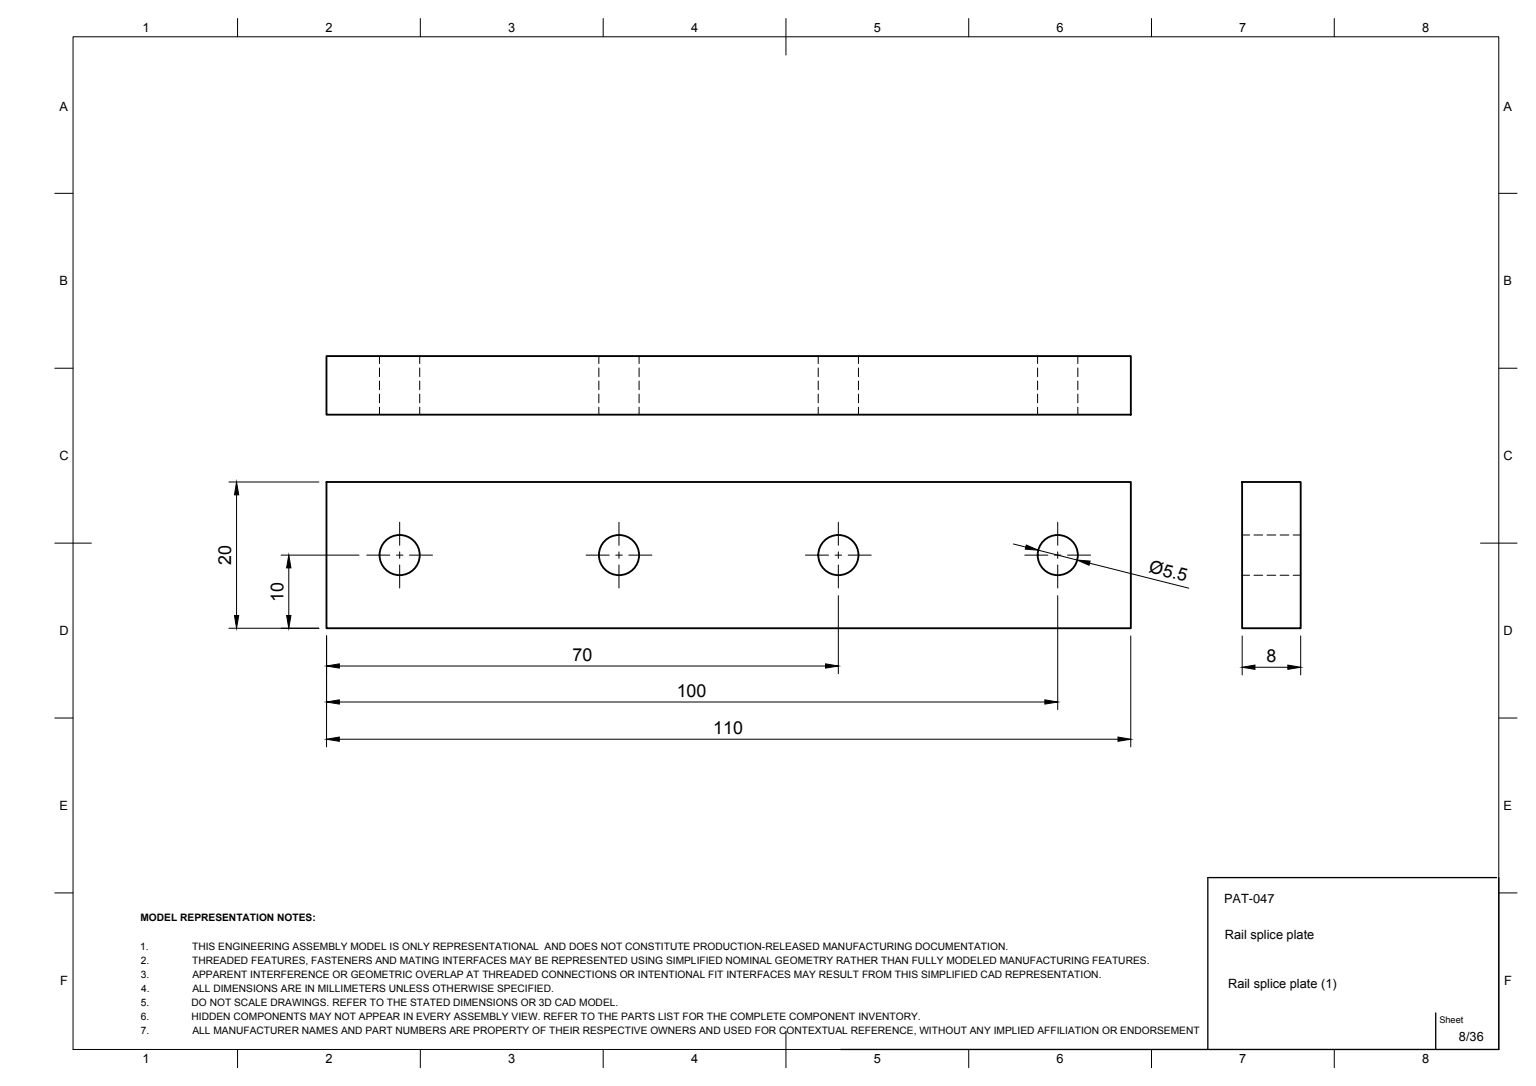
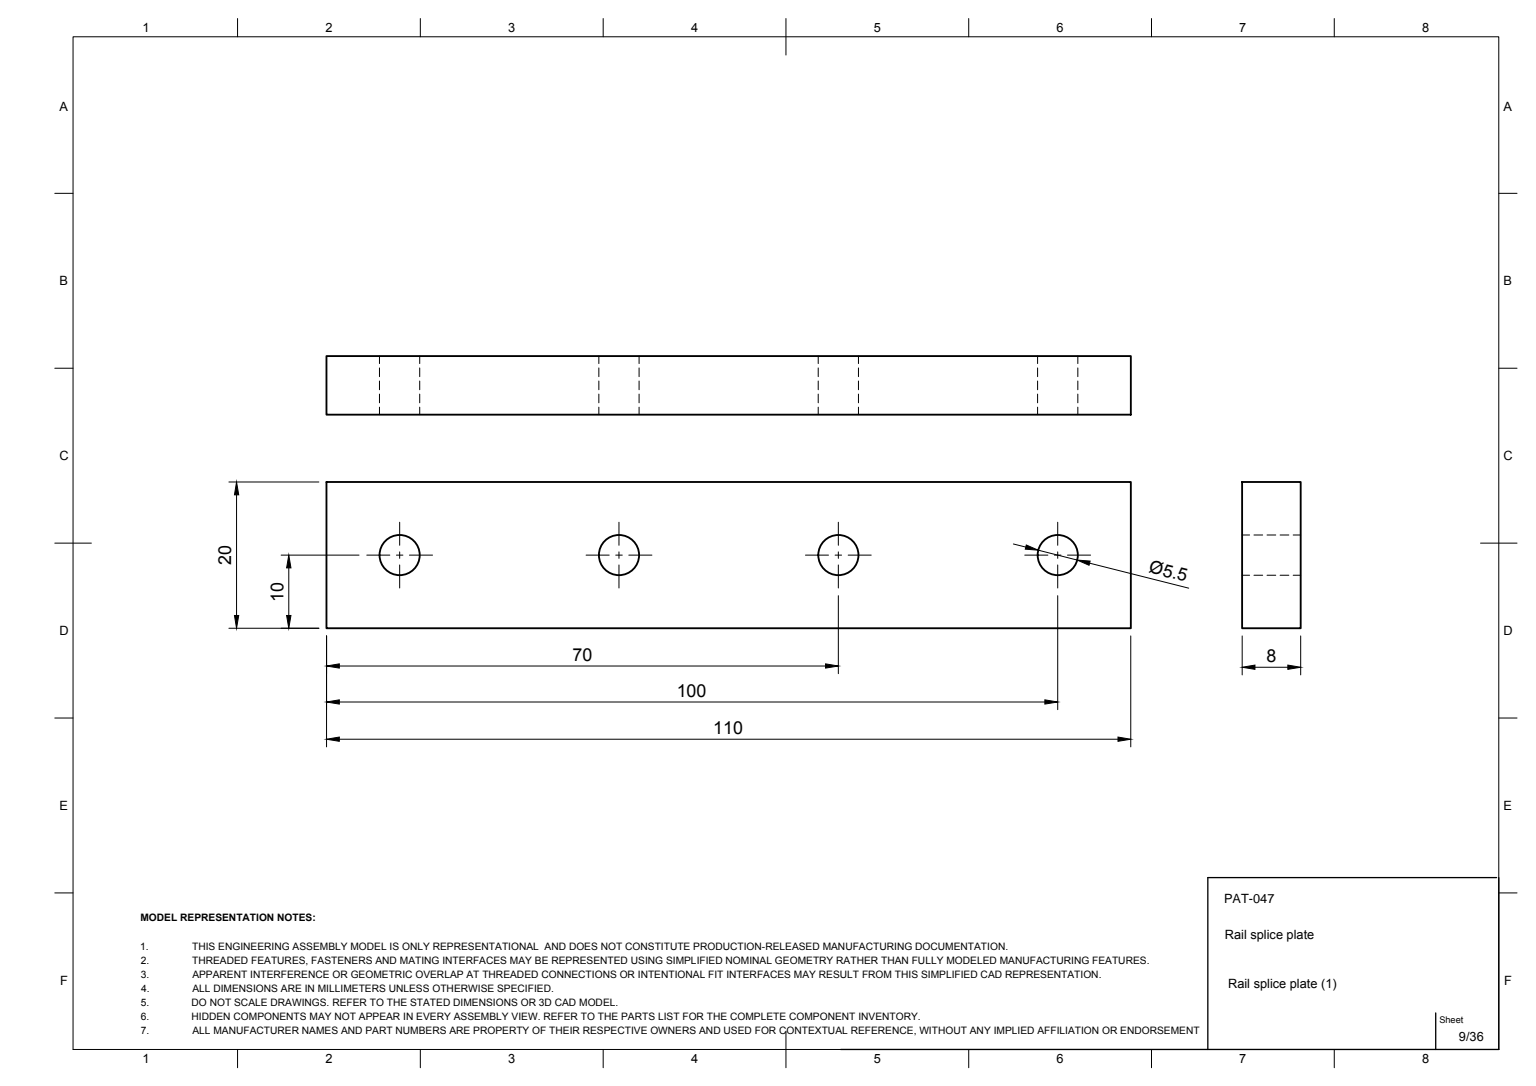
ISO-10303-21;
HEADER;
/* Generated by software containing ST-Developer
 * from STEP Tools, Inc. (www.steptools.com) 
 */

FILE_DESCRIPTION(
/* description */ ('Gravity roller conveyor section'),
/* implementation_level */ '2;1');

FILE_NAME(
/* name */ 'Rail splice plate.step',
/* time_stamp */ '2026-11-02T07:43:02-08:00',
/* author */ (''),
/* organization */ (''),
/* preprocessor_version */ 'ST-DEVELOPER v20.2',
/* originating_system */ 'Autodesk Translation Framework v15.17.0.0',
/* authorisation */ '');

FILE_SCHEMA (('AUTOMOTIVE_DESIGN { 1 0 10303 214 3 1 1 }'));
ENDSEC;

DATA;
#10=MECHANICAL_DESIGN_GEOMETRIC_PRESENTATION_REPRESENTATION('',(#529),#13821);
#461=SHAPE_REPRESENTATION_RELATIONSHIP('SRR','None',#13998,#495);
#495=ADVANCED_BREP_SHAPE_REPRESENTATION('',(#571),#13785);
#529=STYLED_ITEM('',(#14191),#571);
#571=MANIFOLD_SOLID_BREP('Body1',#7627);
#609=FACE_BOUND('',#1431,.T.);
#610=FACE_BOUND('',#1432,.T.);
#611=FACE_BOUND('',#1433,.T.);
#612=FACE_BOUND('',#1434,.T.);
#613=FACE_BOUND('',#1437,.T.);
#614=FACE_BOUND('',#1438,.T.);
#615=FACE_BOUND('',#1439,.T.);
#616=FACE_BOUND('',#1440,.T.);
#702=PLANE('',#8063);
#703=PLANE('',#8064);
#704=PLANE('',#8065);
#705=PLANE('',#8066);
#706=PLANE('',#8067);
#707=PLANE('',#8068);
#1007=FACE_OUTER_BOUND('',#1426,.T.);
#1008=FACE_OUTER_BOUND('',#1427,.T.);
#1009=FACE_OUTER_BOUND('',#1428,.T.);
#1010=FACE_OUTER_BOUND('',#1429,.T.);
#1011=FACE_OUTER_BOUND('',#1430,.T.);
#1012=FACE_OUTER_BOUND('',#1435,.T.);
#1013=FACE_OUTER_BOUND('',#1436,.T.);
#1014=FACE_OUTER_BOUND('',#1441,.T.);
#1015=FACE_OUTER_BOUND('',#1442,.T.);
#1016=FACE_OUTER_BOUND('',#1443,.T.);
#1426=EDGE_LOOP('',(#5202,#5203,#5204,#5205));
#1427=EDGE_LOOP('',(#5206,#5207,#5208,#5209));
#1428=EDGE_LOOP('',(#5210,#5211,#5212,#5213));
#1429=EDGE_LOOP('',(#5214,#5215,#5216,#5217));
#1430=EDGE_LOOP('',(#5218,#5219,#5220,#5221));
#1431=EDGE_LOOP('',(#5222));
#1432=EDGE_LOOP('',(#5223));
#1433=EDGE_LOOP('',(#5224));
#1434=EDGE_LOOP('',(#5225));
#1435=EDGE_LOOP('',(#5226,#5227,#5228,#5229));
#1436=EDGE_LOOP('',(#5230,#5231,#5232,#5233));
#1437=EDGE_LOOP('',(#5234));
#1438=EDGE_LOOP('',(#5235));
#1439=EDGE_LOOP('',(#5236));
#1440=EDGE_LOOP('',(#5237));
#1441=EDGE_LOOP('',(#5238,#5239,#5240,#5241));
#1442=EDGE_LOOP('',(#5242,#5243,#5244,#5245));
#1443=EDGE_LOOP('',(#5246,#5247,#5248,#5249));
#1938=LINE('',#11080,#2656);
#1939=LINE('',#11086,#2657);
#1940=LINE('',#11092,#2658);
#1941=LINE('',#11098,#2659);
#1942=LINE('',#11103,#2660);
#1943=LINE('',#11105,#2661);
#1944=LINE('',#11107,#2662);
#1945=LINE('',#11108,#2663);
#1946=LINE('',#11111,#2664);
#1947=LINE('',#11113,#2665);
#1948=LINE('',#11114,#2666);
#1949=LINE('',#11117,#2667);
#1950=LINE('',#11119,#2668);
#1951=LINE('',#11120,#2669);
#1952=LINE('',#11122,#2670);
#1953=LINE('',#11123,#2671);
#2656=VECTOR('',#8827,0.274999999999999);
#2657=VECTOR('',#8834,0.274999999999999);
#2658=VECTOR('',#8841,0.274999999999999);
#2659=VECTOR('',#8848,0.274999999999999);
#2660=VECTOR('',#8853,1.);
#2661=VECTOR('',#8854,1.);
#2662=VECTOR('',#8855,1.);
#2663=VECTOR('',#8856,1.);
#2664=VECTOR('',#8859,1.);
#2665=VECTOR('',#8860,1.);
#2666=VECTOR('',#8861,1.);
#2667=VECTOR('',#8864,1.);
#2668=VECTOR('',#8865,1.);
#2669=VECTOR('',#8866,1.);
#2670=VECTOR('',#8869,1.);
#2671=VECTOR('',#8870,1.);
#3374=CIRCLE('',#8052,0.274999999999999);
#3375=CIRCLE('',#8053,0.274999999999999);
#3376=CIRCLE('',#8055,0.274999999999999);
#3377=CIRCLE('',#8056,0.274999999999999);
#3378=CIRCLE('',#8058,0.274999999999999);
#3379=CIRCLE('',#8059,0.274999999999999);
#3380=CIRCLE('',#8061,0.274999999999999);
#3381=CIRCLE('',#8062,0.274999999999999);
#3590=VERTEX_POINT('',#11077);
#3591=VERTEX_POINT('',#11079);
#3592=VERTEX_POINT('',#11083);
#3593=VERTEX_POINT('',#11085);
#3594=VERTEX_POINT('',#11089);
#3595=VERTEX_POINT('',#11091);
#3596=VERTEX_POINT('',#11095);
#3597=VERTEX_POINT('',#11097);
#3598=VERTEX_POINT('',#11101);
#3599=VERTEX_POINT('',#11102);
#3600=VERTEX_POINT('',#11104);
#3601=VERTEX_POINT('',#11106);
#3602=VERTEX_POINT('',#11110);
#3603=VERTEX_POINT('',#11112);
#3604=VERTEX_POINT('',#11116);
#3605=VERTEX_POINT('',#11118);
#4238=EDGE_CURVE('',#3590,#3590,#3374,.T.);
#4239=EDGE_CURVE('',#3590,#3591,#1938,.T.);
#4240=EDGE_CURVE('',#3591,#3591,#3375,.T.);
#4241=EDGE_CURVE('',#3592,#3592,#3376,.T.);
#4242=EDGE_CURVE('',#3592,#3593,#1939,.T.);
#4243=EDGE_CURVE('',#3593,#3593,#3377,.T.);
#4244=EDGE_CURVE('',#3594,#3594,#3378,.T.);
#4245=EDGE_CURVE('',#3594,#3595,#1940,.T.);
#4246=EDGE_CURVE('',#3595,#3595,#3379,.T.);
#4247=EDGE_CURVE('',#3596,#3596,#3380,.T.);
#4248=EDGE_CURVE('',#3596,#3597,#1941,.T.);
#4249=EDGE_CURVE('',#3597,#3597,#3381,.T.);
#4250=EDGE_CURVE('',#3598,#3599,#1942,.T.);
#4251=EDGE_CURVE('',#3599,#3600,#1943,.T.);
#4252=EDGE_CURVE('',#3601,#3600,#1944,.T.);
#4253=EDGE_CURVE('',#3598,#3601,#1945,.T.);
#4254=EDGE_CURVE('',#3602,#3598,#1946,.T.);
#4255=EDGE_CURVE('',#3603,#3601,#1947,.T.);
#4256=EDGE_CURVE('',#3602,#3603,#1948,.T.);
#4257=EDGE_CURVE('',#3604,#3602,#1949,.T.);
#4258=EDGE_CURVE('',#3605,#3603,#1950,.T.);
#4259=EDGE_CURVE('',#3604,#3605,#1951,.T.);
#4260=EDGE_CURVE('',#3599,#3604,#1952,.T.);
#4261=EDGE_CURVE('',#3600,#3605,#1953,.T.);
#5202=ORIENTED_EDGE('',*,*,#4238,.F.);
#5203=ORIENTED_EDGE('',*,*,#4239,.T.);
#5204=ORIENTED_EDGE('',*,*,#4240,.F.);
#5205=ORIENTED_EDGE('',*,*,#4239,.F.);
#5206=ORIENTED_EDGE('',*,*,#4241,.F.);
#5207=ORIENTED_EDGE('',*,*,#4242,.T.);
#5208=ORIENTED_EDGE('',*,*,#4243,.F.);
#5209=ORIENTED_EDGE('',*,*,#4242,.F.);
#5210=ORIENTED_EDGE('',*,*,#4244,.F.);
#5211=ORIENTED_EDGE('',*,*,#4245,.T.);
#5212=ORIENTED_EDGE('',*,*,#4246,.F.);
#5213=ORIENTED_EDGE('',*,*,#4245,.F.);
#5214=ORIENTED_EDGE('',*,*,#4247,.F.);
#5215=ORIENTED_EDGE('',*,*,#4248,.T.);
#5216=ORIENTED_EDGE('',*,*,#4249,.F.);
#5217=ORIENTED_EDGE('',*,*,#4248,.F.);
#5218=ORIENTED_EDGE('',*,*,#4250,.T.);
#5219=ORIENTED_EDGE('',*,*,#4251,.T.);
#5220=ORIENTED_EDGE('',*,*,#4252,.F.);
#5221=ORIENTED_EDGE('',*,*,#4253,.F.);
#5222=ORIENTED_EDGE('',*,*,#4240,.T.);
#5223=ORIENTED_EDGE('',*,*,#4243,.T.);
#5224=ORIENTED_EDGE('',*,*,#4246,.T.);
#5225=ORIENTED_EDGE('',*,*,#4249,.T.);
#5226=ORIENTED_EDGE('',*,*,#4254,.T.);
#5227=ORIENTED_EDGE('',*,*,#4253,.T.);
#5228=ORIENTED_EDGE('',*,*,#4255,.F.);
#5229=ORIENTED_EDGE('',*,*,#4256,.F.);
#5230=ORIENTED_EDGE('',*,*,#4257,.T.);
#5231=ORIENTED_EDGE('',*,*,#4256,.T.);
#5232=ORIENTED_EDGE('',*,*,#4258,.F.);
#5233=ORIENTED_EDGE('',*,*,#4259,.F.);
#5234=ORIENTED_EDGE('',*,*,#4238,.T.);
#5235=ORIENTED_EDGE('',*,*,#4241,.T.);
#5236=ORIENTED_EDGE('',*,*,#4244,.T.);
#5237=ORIENTED_EDGE('',*,*,#4247,.T.);
#5238=ORIENTED_EDGE('',*,*,#4260,.T.);
#5239=ORIENTED_EDGE('',*,*,#4259,.T.);
#5240=ORIENTED_EDGE('',*,*,#4261,.F.);
#5241=ORIENTED_EDGE('',*,*,#4251,.F.);
#5242=ORIENTED_EDGE('',*,*,#4261,.T.);
#5243=ORIENTED_EDGE('',*,*,#4258,.T.);
#5244=ORIENTED_EDGE('',*,*,#4255,.T.);
#5245=ORIENTED_EDGE('',*,*,#4252,.T.);
#5246=ORIENTED_EDGE('',*,*,#4260,.F.);
#5247=ORIENTED_EDGE('',*,*,#4250,.F.);
#5248=ORIENTED_EDGE('',*,*,#4254,.F.);
#5249=ORIENTED_EDGE('',*,*,#4257,.F.);
#7130=CYLINDRICAL_SURFACE('',#8051,0.274999999999999);
#7131=CYLINDRICAL_SURFACE('',#8054,0.274999999999999);
#7132=CYLINDRICAL_SURFACE('',#8057,0.274999999999999);
#7133=CYLINDRICAL_SURFACE('',#8060,0.274999999999999);
#7208=ADVANCED_FACE('',(#1007),#7130,.F.);
#7209=ADVANCED_FACE('',(#1008),#7131,.F.);
#7210=ADVANCED_FACE('',(#1009),#7132,.F.);
#7211=ADVANCED_FACE('',(#1010),#7133,.F.);
#7212=ADVANCED_FACE('',(#1011,#609,#610,#611,#612),#702,.T.);
#7213=ADVANCED_FACE('',(#1012),#703,.T.);
#7214=ADVANCED_FACE('',(#1013,#613,#614,#615,#616),#704,.T.);
#7215=ADVANCED_FACE('',(#1014),#705,.T.);
#7216=ADVANCED_FACE('',(#1015),#706,.T.);
#7217=ADVANCED_FACE('',(#1016),#707,.F.);
#7627=CLOSED_SHELL('',(#7208,#7209,#7210,#7211,#7212,#7213,#7214,#7215,
#7216,#7217));
#8050=AXIS2_PLACEMENT_3D('',#11075,#8821,#8822);
#8051=AXIS2_PLACEMENT_3D('',#11076,#8823,#8824);
#8052=AXIS2_PLACEMENT_3D('',#11078,#8825,#8826);
#8053=AXIS2_PLACEMENT_3D('',#11081,#8828,#8829);
#8054=AXIS2_PLACEMENT_3D('',#11082,#8830,#8831);
#8055=AXIS2_PLACEMENT_3D('',#11084,#8832,#8833);
#8056=AXIS2_PLACEMENT_3D('',#11087,#8835,#8836);
#8057=AXIS2_PLACEMENT_3D('',#11088,#8837,#8838);
#8058=AXIS2_PLACEMENT_3D('',#11090,#8839,#8840);
#8059=AXIS2_PLACEMENT_3D('',#11093,#8842,#8843);
#8060=AXIS2_PLACEMENT_3D('',#11094,#8844,#8845);
#8061=AXIS2_PLACEMENT_3D('',#11096,#8846,#8847);
#8062=AXIS2_PLACEMENT_3D('',#11099,#8849,#8850);
#8063=AXIS2_PLACEMENT_3D('',#11100,#8851,#8852);
#8064=AXIS2_PLACEMENT_3D('',#11109,#8857,#8858);
#8065=AXIS2_PLACEMENT_3D('',#11115,#8862,#8863);
#8066=AXIS2_PLACEMENT_3D('',#11121,#8867,#8868);
#8067=AXIS2_PLACEMENT_3D('',#11124,#8871,#8872);
#8068=AXIS2_PLACEMENT_3D('',#11125,#8873,#8874);
#8821=DIRECTION('axis',(0.,0.,1.));
#8822=DIRECTION('refdir',(1.,0.,0.));
#8823=DIRECTION('center_axis',(0.,1.,0.));
#8824=DIRECTION('ref_axis',(1.,0.,0.));
#8825=DIRECTION('center_axis',(0.,1.,0.));
#8826=DIRECTION('ref_axis',(1.,0.,0.));
#8827=DIRECTION('',(0.,1.,0.));
#8828=DIRECTION('center_axis',(0.,-1.,0.));
#8829=DIRECTION('ref_axis',(1.,0.,0.));
#8830=DIRECTION('center_axis',(0.,1.,0.));
#8831=DIRECTION('ref_axis',(1.,0.,0.));
#8832=DIRECTION('center_axis',(0.,1.,0.));
#8833=DIRECTION('ref_axis',(1.,0.,0.));
#8834=DIRECTION('',(0.,1.,0.));
#8835=DIRECTION('center_axis',(0.,-1.,0.));
#8836=DIRECTION('ref_axis',(1.,0.,0.));
#8837=DIRECTION('center_axis',(0.,1.,0.));
#8838=DIRECTION('ref_axis',(1.,0.,0.));
#8839=DIRECTION('center_axis',(0.,1.,0.));
#8840=DIRECTION('ref_axis',(1.,0.,0.));
#8841=DIRECTION('',(0.,1.,0.));
#8842=DIRECTION('center_axis',(0.,-1.,0.));
#8843=DIRECTION('ref_axis',(1.,0.,0.));
#8844=DIRECTION('center_axis',(0.,1.,0.));
#8845=DIRECTION('ref_axis',(1.,0.,0.));
#8846=DIRECTION('center_axis',(0.,1.,0.));
#8847=DIRECTION('ref_axis',(1.,0.,0.));
#8848=DIRECTION('',(0.,1.,0.));
#8849=DIRECTION('center_axis',(0.,-1.,0.));
#8850=DIRECTION('ref_axis',(1.,0.,0.));
#8851=DIRECTION('center_axis',(0.,1.,0.));
#8852=DIRECTION('ref_axis',(-1.,0.,0.));
#8853=DIRECTION('',(-1.,0.,0.));
#8854=DIRECTION('',(0.,0.,1.));
#8855=DIRECTION('',(-1.,0.,0.));
#8856=DIRECTION('',(0.,0.,1.));
#8857=DIRECTION('center_axis',(1.,0.,0.));
#8858=DIRECTION('ref_axis',(0.,1.,0.));
#8859=DIRECTION('',(0.,1.,0.));
#8860=DIRECTION('',(0.,1.,0.));
#8861=DIRECTION('',(0.,0.,1.));
#8862=DIRECTION('center_axis',(0.,-1.,0.));
#8863=DIRECTION('ref_axis',(1.,0.,0.));
#8864=DIRECTION('',(1.,0.,0.));
#8865=DIRECTION('',(1.,0.,0.));
#8866=DIRECTION('',(0.,0.,1.));
#8867=DIRECTION('center_axis',(-1.,0.,0.));
#8868=DIRECTION('ref_axis',(0.,-1.,0.));
#8869=DIRECTION('',(0.,-1.,0.));
#8870=DIRECTION('',(0.,-1.,0.));
#8871=DIRECTION('center_axis',(0.,0.,1.));
#8872=DIRECTION('ref_axis',(1.,0.,0.));
#8873=DIRECTION('center_axis',(0.,0.,1.));
#8874=DIRECTION('ref_axis',(1.,0.,0.));
#11075=CARTESIAN_POINT('',(0.,0.,0.));
#11076=CARTESIAN_POINT('Origin',(42.,-3.9,5.));
#11077=CARTESIAN_POINT('',(41.725,-3.8,5.));
#11078=CARTESIAN_POINT('Origin',(42.,-3.8,5.));
#11079=CARTESIAN_POINT('',(41.725,-3.,5.));
#11080=CARTESIAN_POINT('',(41.725,-3.9,5.));
#11081=CARTESIAN_POINT('Origin',(42.,-3.,5.));
#11082=CARTESIAN_POINT('Origin',(39.,-3.9,5.));
#11083=CARTESIAN_POINT('',(38.725,-3.8,5.));
#11084=CARTESIAN_POINT('Origin',(39.,-3.8,5.));
#11085=CARTESIAN_POINT('',(38.725,-3.,5.));
#11086=CARTESIAN_POINT('',(38.725,-3.9,5.));
#11087=CARTESIAN_POINT('Origin',(39.,-3.,5.));
#11088=CARTESIAN_POINT('Origin',(36.,-3.9,5.));
#11089=CARTESIAN_POINT('',(35.725,-3.8,5.));
#11090=CARTESIAN_POINT('Origin',(36.,-3.8,5.));
#11091=CARTESIAN_POINT('',(35.725,-3.,5.));
#11092=CARTESIAN_POINT('',(35.725,-3.9,5.));
#11093=CARTESIAN_POINT('Origin',(36.,-3.,5.));
#11094=CARTESIAN_POINT('Origin',(45.,-3.9,5.));
#11095=CARTESIAN_POINT('',(44.725,-3.8,5.));
#11096=CARTESIAN_POINT('Origin',(45.,-3.8,5.));
#11097=CARTESIAN_POINT('',(44.725,-3.,5.));
#11098=CARTESIAN_POINT('',(44.725,-3.9,5.));
#11099=CARTESIAN_POINT('Origin',(45.,-3.,5.));
#11100=CARTESIAN_POINT('Origin',(46.,-3.,4.));
#11101=CARTESIAN_POINT('',(46.,-3.,4.));
#11102=CARTESIAN_POINT('',(35.,-3.,4.));
#11103=CARTESIAN_POINT('',(46.,-3.,4.));
#11104=CARTESIAN_POINT('',(35.,-3.,6.));
#11105=CARTESIAN_POINT('',(35.,-3.,4.));
#11106=CARTESIAN_POINT('',(46.,-3.,6.));
#11107=CARTESIAN_POINT('',(46.,-3.,6.));
#11108=CARTESIAN_POINT('',(46.,-3.,4.));
#11109=CARTESIAN_POINT('Origin',(46.,-3.8,4.));
#11110=CARTESIAN_POINT('',(46.,-3.8,4.));
#11111=CARTESIAN_POINT('',(46.,-3.8,4.));
#11112=CARTESIAN_POINT('',(46.,-3.8,6.));
#11113=CARTESIAN_POINT('',(46.,-3.8,6.));
#11114=CARTESIAN_POINT('',(46.,-3.8,4.));
#11115=CARTESIAN_POINT('Origin',(35.,-3.8,4.));
#11116=CARTESIAN_POINT('',(35.,-3.8,4.));
#11117=CARTESIAN_POINT('',(35.,-3.8,4.));
#11118=CARTESIAN_POINT('',(35.,-3.8,6.));
#11119=CARTESIAN_POINT('',(35.,-3.8,6.));
#11120=CARTESIAN_POINT('',(35.,-3.8,4.));
#11121=CARTESIAN_POINT('Origin',(35.,-3.,4.));
#11122=CARTESIAN_POINT('',(35.,-3.,4.));
#11123=CARTESIAN_POINT('',(35.,-3.,6.));
#11124=CARTESIAN_POINT('Origin',(40.5,-3.4,6.));
#11125=CARTESIAN_POINT('Origin',(40.5,-3.4,4.));
#13746=UNCERTAINTY_MEASURE_WITH_UNIT(LENGTH_MEASURE(0.001),#13822,
'DISTANCE_ACCURACY_VALUE',
'Maximum model space distance between geometric entities at asserted c
onnectivities');
#13782=UNCERTAINTY_MEASURE_WITH_UNIT(LENGTH_MEASURE(0.001),#13822,
'DISTANCE_ACCURACY_VALUE',
'Maximum model space distance between geometric entities at asserted c
onnectivities');
#13785=(
GEOMETRIC_REPRESENTATION_CONTEXT(3)
GLOBAL_UNCERTAINTY_ASSIGNED_CONTEXT((#13746))
GLOBAL_UNIT_ASSIGNED_CONTEXT((#13822,#13824,#13825))
REPRESENTATION_CONTEXT('','3D')
);
#13821=(
GEOMETRIC_REPRESENTATION_CONTEXT(3)
GLOBAL_UNCERTAINTY_ASSIGNED_CONTEXT((#13782))
GLOBAL_UNIT_ASSIGNED_CONTEXT((#13822,#13824,#13825))
REPRESENTATION_CONTEXT('','3D')
);
#13822=(
LENGTH_UNIT()
NAMED_UNIT(*)
SI_UNIT(.CENTI.,.METRE.)
);
#13824=(
NAMED_UNIT(*)
PLANE_ANGLE_UNIT()
SI_UNIT($,.RADIAN.)
);
#13825=(
NAMED_UNIT(*)
SI_UNIT($,.STERADIAN.)
SOLID_ANGLE_UNIT()
);
#13828=SHAPE_DEFINITION_REPRESENTATION(#13866,#13998);
#13866=PRODUCT_DEFINITION_SHAPE('',$,#14037);
#13998=SHAPE_REPRESENTATION('',(#8050),#13785);
#14034=PRODUCT_DEFINITION_CONTEXT('part definition',#14150,'design');
#14037=PRODUCT_DEFINITION('Rail splice plate','Rail splice plate',#14075,
#14034);
#14075=PRODUCT_DEFINITION_FORMATION('',$,#14154);
#14150=APPLICATION_CONTEXT(
'Core Data for Automotive Mechanical Design Process');
#14151=PRODUCT_CONTEXT('part definition',#14150,'mechanical');
#14154=PRODUCT('Rail splice plate','Rail splice plate',
'Rail splice plate',(#14151));
#14191=PRESENTATION_STYLE_ASSIGNMENT((#14196));
#14196=SURFACE_STYLE_USAGE(.BOTH.,#14201);
#14201=SURFACE_SIDE_STYLE('',(#14206));
#14206=SURFACE_STYLE_FILL_AREA(#14211);
#14211=FILL_AREA_STYLE('CAD Library Painted - Steel gray',(#14216));
#14216=FILL_AREA_STYLE_COLOUR('CAD Library Painted - Steel gray',#14221);
#14221=COLOUR_RGB('CAD Library Painted - Steel gray',0.592156862745098,
0.631372549019608,0.67843137254902);
ENDSEC;
END-ISO-10303-21;
